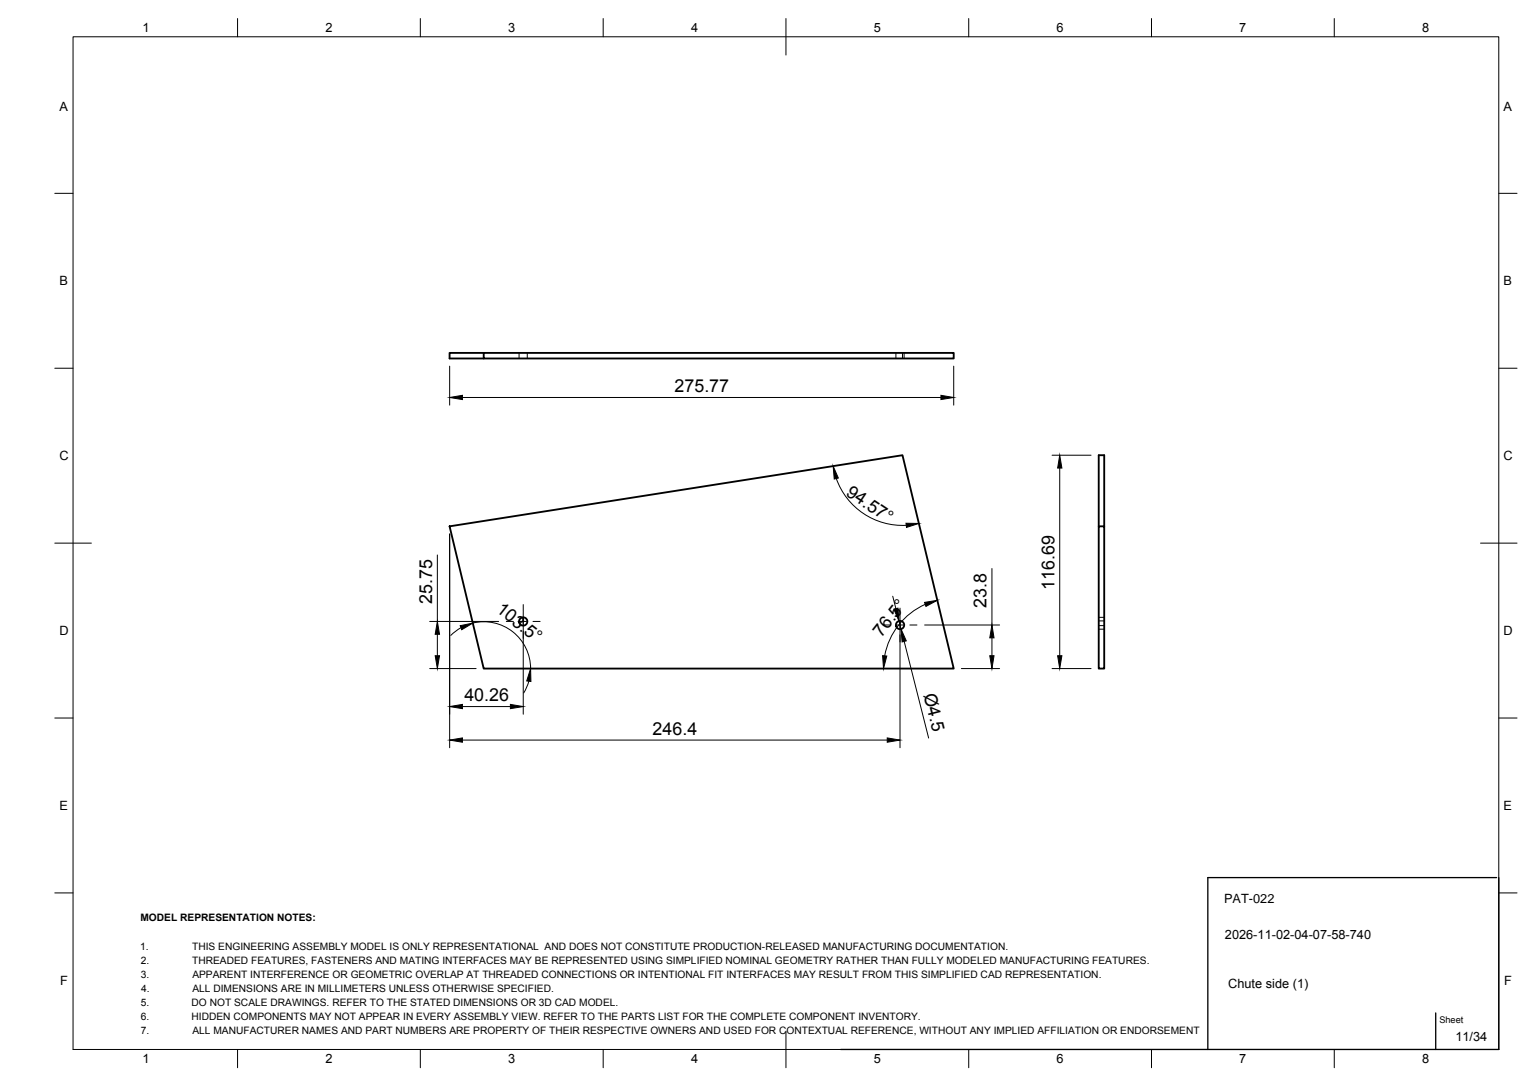
ISO-10303-21;
HEADER;
/* Generated by software containing ST-Developer
 * from STEP Tools, Inc. (www.steptools.com) 
 */

FILE_DESCRIPTION(
/* description */ ('Chute with adjustable gate'),
/* implementation_level */ '2;1');

FILE_NAME(
/* name */ 'Chute side (1).step',
/* time_stamp */ '2026-10-27T10:52:28-07:00',
/* author */ (''),
/* organization */ (''),
/* preprocessor_version */ 'ST-DEVELOPER v20.2',
/* originating_system */ 'Autodesk Translation Framework v15.17.0.0',
/* authorisation */ '');

FILE_SCHEMA (('AUTOMOTIVE_DESIGN { 1 0 10303 214 3 1 1 }'));
ENDSEC;

DATA;
#10=MECHANICAL_DESIGN_GEOMETRIC_PRESENTATION_REPRESENTATION('',(#420),#13094);
#356=SHAPE_REPRESENTATION_RELATIONSHIP('SRR','None',#13257,#388);
#388=ADVANCED_BREP_SHAPE_REPRESENTATION('',(#452),#13066);
#420=STYLED_ITEM('',(#13509),#452);
#452=MANIFOLD_SOLID_BREP('Body1',#7603);
#496=FACE_BOUND('',#1408,.T.);
#497=FACE_BOUND('',#1409,.T.);
#498=FACE_BOUND('',#1411,.T.);
#499=FACE_BOUND('',#1412,.T.);
#630=PLANE('',#8071);
#631=PLANE('',#8072);
#632=PLANE('',#8073);
#633=PLANE('',#8074);
#634=PLANE('',#8075);
#635=PLANE('',#8076);
#964=FACE_OUTER_BOUND('',#1401,.T.);
#965=FACE_OUTER_BOUND('',#1402,.T.);
#966=FACE_OUTER_BOUND('',#1403,.T.);
#967=FACE_OUTER_BOUND('',#1404,.T.);
#968=FACE_OUTER_BOUND('',#1405,.T.);
#969=FACE_OUTER_BOUND('',#1406,.T.);
#970=FACE_OUTER_BOUND('',#1407,.T.);
#971=FACE_OUTER_BOUND('',#1410,.T.);
#1401=EDGE_LOOP('',(#5414,#5415,#5416,#5417));
#1402=EDGE_LOOP('',(#5418,#5419,#5420,#5421));
#1403=EDGE_LOOP('',(#5422,#5423,#5424,#5425));
#1404=EDGE_LOOP('',(#5426,#5427,#5428,#5429));
#1405=EDGE_LOOP('',(#5430,#5431,#5432,#5433));
#1406=EDGE_LOOP('',(#5434,#5435,#5436,#5437));
#1407=EDGE_LOOP('',(#5438,#5439,#5440,#5441));
#1408=EDGE_LOOP('',(#5442));
#1409=EDGE_LOOP('',(#5443));
#1410=EDGE_LOOP('',(#5444,#5445,#5446,#5447));
#1411=EDGE_LOOP('',(#5448));
#1412=EDGE_LOOP('',(#5449));
#1954=LINE('',#11152,#2731);
#1955=LINE('',#11158,#2732);
#1956=LINE('',#11163,#2733);
#1957=LINE('',#11165,#2734);
#1958=LINE('',#11167,#2735);
#1959=LINE('',#11168,#2736);
#1960=LINE('',#11171,#2737);
#1961=LINE('',#11173,#2738);
#1962=LINE('',#11174,#2739);
#1963=LINE('',#11177,#2740);
#1964=LINE('',#11179,#2741);
#1965=LINE('',#11180,#2742);
#1966=LINE('',#11182,#2743);
#1967=LINE('',#11183,#2744);
#2731=VECTOR('',#8954,0.225);
#2732=VECTOR('',#8961,0.225000000000001);
#2733=VECTOR('',#8966,1.);
#2734=VECTOR('',#8967,1.);
#2735=VECTOR('',#8968,1.);
#2736=VECTOR('',#8969,1.);
#2737=VECTOR('',#8972,1.);
#2738=VECTOR('',#8973,1.);
#2739=VECTOR('',#8974,1.);
#2740=VECTOR('',#8977,1.);
#2741=VECTOR('',#8978,1.);
#2742=VECTOR('',#8979,1.);
#2743=VECTOR('',#8982,1.);
#2744=VECTOR('',#8983,1.);
#3434=CIRCLE('',#8066,0.225);
#3435=CIRCLE('',#8067,0.225);
#3436=CIRCLE('',#8069,0.225000000000001);
#3437=CIRCLE('',#8070,0.225000000000001);
#3669=VERTEX_POINT('',#11149);
#3670=VERTEX_POINT('',#11151);
#3671=VERTEX_POINT('',#11155);
#3672=VERTEX_POINT('',#11157);
#3673=VERTEX_POINT('',#11161);
#3674=VERTEX_POINT('',#11162);
#3675=VERTEX_POINT('',#11164);
#3676=VERTEX_POINT('',#11166);
#3677=VERTEX_POINT('',#11170);
#3678=VERTEX_POINT('',#11172);
#3679=VERTEX_POINT('',#11176);
#3680=VERTEX_POINT('',#11178);
#4340=EDGE_CURVE('',#3669,#3669,#3434,.T.);
#4341=EDGE_CURVE('',#3669,#3670,#1954,.T.);
#4342=EDGE_CURVE('',#3670,#3670,#3435,.T.);
#4343=EDGE_CURVE('',#3671,#3671,#3436,.T.);
#4344=EDGE_CURVE('',#3671,#3672,#1955,.T.);
#4345=EDGE_CURVE('',#3672,#3672,#3437,.T.);
#4346=EDGE_CURVE('',#3673,#3674,#1956,.T.);
#4347=EDGE_CURVE('',#3673,#3675,#1957,.T.);
#4348=EDGE_CURVE('',#3676,#3675,#1958,.T.);
#4349=EDGE_CURVE('',#3674,#3676,#1959,.T.);
#4350=EDGE_CURVE('',#3674,#3677,#1960,.T.);
#4351=EDGE_CURVE('',#3678,#3676,#1961,.T.);
#4352=EDGE_CURVE('',#3677,#3678,#1962,.T.);
#4353=EDGE_CURVE('',#3677,#3679,#1963,.T.);
#4354=EDGE_CURVE('',#3680,#3678,#1964,.T.);
#4355=EDGE_CURVE('',#3679,#3680,#1965,.T.);
#4356=EDGE_CURVE('',#3679,#3673,#1966,.T.);
#4357=EDGE_CURVE('',#3675,#3680,#1967,.T.);
#5414=ORIENTED_EDGE('',*,*,#4340,.F.);
#5415=ORIENTED_EDGE('',*,*,#4341,.T.);
#5416=ORIENTED_EDGE('',*,*,#4342,.F.);
#5417=ORIENTED_EDGE('',*,*,#4341,.F.);
#5418=ORIENTED_EDGE('',*,*,#4343,.F.);
#5419=ORIENTED_EDGE('',*,*,#4344,.T.);
#5420=ORIENTED_EDGE('',*,*,#4345,.F.);
#5421=ORIENTED_EDGE('',*,*,#4344,.F.);
#5422=ORIENTED_EDGE('',*,*,#4346,.F.);
#5423=ORIENTED_EDGE('',*,*,#4347,.T.);
#5424=ORIENTED_EDGE('',*,*,#4348,.F.);
#5425=ORIENTED_EDGE('',*,*,#4349,.F.);
#5426=ORIENTED_EDGE('',*,*,#4350,.F.);
#5427=ORIENTED_EDGE('',*,*,#4349,.T.);
#5428=ORIENTED_EDGE('',*,*,#4351,.F.);
#5429=ORIENTED_EDGE('',*,*,#4352,.F.);
#5430=ORIENTED_EDGE('',*,*,#4353,.F.);
#5431=ORIENTED_EDGE('',*,*,#4352,.T.);
#5432=ORIENTED_EDGE('',*,*,#4354,.F.);
#5433=ORIENTED_EDGE('',*,*,#4355,.F.);
#5434=ORIENTED_EDGE('',*,*,#4356,.F.);
#5435=ORIENTED_EDGE('',*,*,#4355,.T.);
#5436=ORIENTED_EDGE('',*,*,#4357,.F.);
#5437=ORIENTED_EDGE('',*,*,#4347,.F.);
#5438=ORIENTED_EDGE('',*,*,#4357,.T.);
#5439=ORIENTED_EDGE('',*,*,#4354,.T.);
#5440=ORIENTED_EDGE('',*,*,#4351,.T.);
#5441=ORIENTED_EDGE('',*,*,#4348,.T.);
#5442=ORIENTED_EDGE('',*,*,#4342,.T.);
#5443=ORIENTED_EDGE('',*,*,#4345,.T.);
#5444=ORIENTED_EDGE('',*,*,#4356,.T.);
#5445=ORIENTED_EDGE('',*,*,#4346,.T.);
#5446=ORIENTED_EDGE('',*,*,#4350,.T.);
#5447=ORIENTED_EDGE('',*,*,#4353,.T.);
#5448=ORIENTED_EDGE('',*,*,#4340,.T.);
#5449=ORIENTED_EDGE('',*,*,#4343,.T.);
#7116=CYLINDRICAL_SURFACE('',#8065,0.225);
#7117=CYLINDRICAL_SURFACE('',#8068,0.225000000000001);
#7232=ADVANCED_FACE('',(#964),#7116,.F.);
#7233=ADVANCED_FACE('',(#965),#7117,.F.);
#7234=ADVANCED_FACE('',(#966),#630,.T.);
#7235=ADVANCED_FACE('',(#967),#631,.T.);
#7236=ADVANCED_FACE('',(#968),#632,.T.);
#7237=ADVANCED_FACE('',(#969),#633,.T.);
#7238=ADVANCED_FACE('',(#970,#496,#497),#634,.T.);
#7239=ADVANCED_FACE('',(#971,#498,#499),#635,.F.);
#7603=CLOSED_SHELL('',(#7232,#7233,#7234,#7235,#7236,#7237,#7238,#7239));
#8064=AXIS2_PLACEMENT_3D('',#11147,#8948,#8949);
#8065=AXIS2_PLACEMENT_3D('',#11148,#8950,#8951);
#8066=AXIS2_PLACEMENT_3D('',#11150,#8952,#8953);
#8067=AXIS2_PLACEMENT_3D('',#11153,#8955,#8956);
#8068=AXIS2_PLACEMENT_3D('',#11154,#8957,#8958);
#8069=AXIS2_PLACEMENT_3D('',#11156,#8959,#8960);
#8070=AXIS2_PLACEMENT_3D('',#11159,#8962,#8963);
#8071=AXIS2_PLACEMENT_3D('',#11160,#8964,#8965);
#8072=AXIS2_PLACEMENT_3D('',#11169,#8970,#8971);
#8073=AXIS2_PLACEMENT_3D('',#11175,#8975,#8976);
#8074=AXIS2_PLACEMENT_3D('',#11181,#8980,#8981);
#8075=AXIS2_PLACEMENT_3D('',#11184,#8984,#8985);
#8076=AXIS2_PLACEMENT_3D('',#11185,#8986,#8987);
#8948=DIRECTION('axis',(0.,0.,1.));
#8949=DIRECTION('refdir',(1.,0.,0.));
#8950=DIRECTION('center_axis',(0.,1.,0.));
#8951=DIRECTION('ref_axis',(1.,0.,0.));
#8952=DIRECTION('center_axis',(0.,1.,0.));
#8953=DIRECTION('ref_axis',(1.,0.,0.));
#8954=DIRECTION('',(0.,1.,0.));
#8955=DIRECTION('center_axis',(0.,-1.,0.));
#8956=DIRECTION('ref_axis',(1.,0.,0.));
#8957=DIRECTION('center_axis',(0.,1.,0.));
#8958=DIRECTION('ref_axis',(1.,0.,0.));
#8959=DIRECTION('center_axis',(0.,1.,0.));
#8960=DIRECTION('ref_axis',(1.,0.,0.));
#8961=DIRECTION('',(0.,1.,0.));
#8962=DIRECTION('center_axis',(0.,-1.,0.));
#8963=DIRECTION('ref_axis',(1.,0.,0.));
#8964=DIRECTION('center_axis',(-1.,0.,0.));
#8965=DIRECTION('ref_axis',(0.,0.,1.));
#8966=DIRECTION('',(0.,0.,-1.));
#8967=DIRECTION('',(0.,1.,0.));
#8968=DIRECTION('',(0.,0.,1.));
#8969=DIRECTION('',(0.,1.,0.));
#8970=DIRECTION('center_axis',(0.233372952475324,0.,-0.972387301980517));
#8971=DIRECTION('ref_axis',(-0.972387301980517,0.,-0.233372952475324));
#8972=DIRECTION('',(0.972387301980517,0.,0.233372952475324));
#8973=DIRECTION('',(-0.972387301980517,0.,-0.233372952475324));
#8974=DIRECTION('',(0.,1.,0.));
#8975=DIRECTION('center_axis',(1.,0.,0.));
#8976=DIRECTION('ref_axis',(0.,0.,-1.));
#8977=DIRECTION('',(0.,0.,1.));
#8978=DIRECTION('',(0.,0.,-1.));
#8979=DIRECTION('',(0.,1.,0.));
#8980=DIRECTION('center_axis',(-0.07974522228289,0.,0.996815278536125));
#8981=DIRECTION('ref_axis',(0.996815278536125,0.,0.07974522228289));
#8982=DIRECTION('',(-0.996815278536125,0.,-0.07974522228289));
#8983=DIRECTION('',(0.996815278536125,0.,0.07974522228289));
#8984=DIRECTION('center_axis',(0.,1.,0.));
#8985=DIRECTION('ref_axis',(0.,0.,1.));
#8986=DIRECTION('center_axis',(0.,1.,0.));
#8987=DIRECTION('ref_axis',(1.,0.,0.));
#11147=CARTESIAN_POINT('',(0.,0.,0.));
#11148=CARTESIAN_POINT('Origin',(2.3,7.4,7.));
#11149=CARTESIAN_POINT('',(2.075,7.5,7.));
#11150=CARTESIAN_POINT('Origin',(2.3,7.5,7.));
#11151=CARTESIAN_POINT('',(2.075,7.8,7.));
#11152=CARTESIAN_POINT('',(2.075,7.4,7.));
#11153=CARTESIAN_POINT('Origin',(2.3,7.8,7.));
#11154=CARTESIAN_POINT('Origin',(22.3,7.4,12.));
#11155=CARTESIAN_POINT('',(22.075,7.5,12.));
#11156=CARTESIAN_POINT('Origin',(22.3,7.5,12.));
#11157=CARTESIAN_POINT('',(22.075,7.8,12.));
#11158=CARTESIAN_POINT('',(22.075,7.4,12.));
#11159=CARTESIAN_POINT('Origin',(22.3,7.8,12.));
#11160=CARTESIAN_POINT('Origin',(0.,7.5,4.));
#11161=CARTESIAN_POINT('',(0.,7.5,16.));
#11162=CARTESIAN_POINT('',(0.,7.5,4.));
#11163=CARTESIAN_POINT('',(0.,7.5,16.));
#11164=CARTESIAN_POINT('',(0.,7.8,16.));
#11165=CARTESIAN_POINT('',(0.,7.5,16.));
#11166=CARTESIAN_POINT('',(0.,7.8,4.));
#11167=CARTESIAN_POINT('',(0.,7.8,16.));
#11168=CARTESIAN_POINT('',(0.,7.5,4.));
#11169=CARTESIAN_POINT('Origin',(25.,7.5,10.));
#11170=CARTESIAN_POINT('',(25.,7.5,10.));
#11171=CARTESIAN_POINT('',(0.,7.5,4.));
#11172=CARTESIAN_POINT('',(25.,7.8,10.));
#11173=CARTESIAN_POINT('',(0.,7.8,4.));
#11174=CARTESIAN_POINT('',(25.,7.5,10.));
#11175=CARTESIAN_POINT('Origin',(25.,7.5,18.));
#11176=CARTESIAN_POINT('',(25.,7.5,18.));
#11177=CARTESIAN_POINT('',(25.,7.5,10.));
#11178=CARTESIAN_POINT('',(25.,7.8,18.));
#11179=CARTESIAN_POINT('',(25.,7.8,10.));
#11180=CARTESIAN_POINT('',(25.,7.5,18.));
#11181=CARTESIAN_POINT('Origin',(0.,7.5,16.));
#11182=CARTESIAN_POINT('',(25.,7.5,18.));
#11183=CARTESIAN_POINT('',(25.,7.8,18.));
#11184=CARTESIAN_POINT('Origin',(12.5,7.8,11.));
#11185=CARTESIAN_POINT('Origin',(12.5,7.5,11.));
#13029=UNCERTAINTY_MEASURE_WITH_UNIT(LENGTH_MEASURE(0.001),#13095,
'DISTANCE_ACCURACY_VALUE',
'Maximum model space distance between geometric entities at asserted c
onnectivities');
#13057=UNCERTAINTY_MEASURE_WITH_UNIT(LENGTH_MEASURE(0.001),#13095,
'DISTANCE_ACCURACY_VALUE',
'Maximum model space distance between geometric entities at asserted c
onnectivities');
#13066=(
GEOMETRIC_REPRESENTATION_CONTEXT(3)
GLOBAL_UNCERTAINTY_ASSIGNED_CONTEXT((#13029))
GLOBAL_UNIT_ASSIGNED_CONTEXT((#13095,#13097,#13098))
REPRESENTATION_CONTEXT('','3D')
);
#13094=(
GEOMETRIC_REPRESENTATION_CONTEXT(3)
GLOBAL_UNCERTAINTY_ASSIGNED_CONTEXT((#13057))
GLOBAL_UNIT_ASSIGNED_CONTEXT((#13095,#13097,#13098))
REPRESENTATION_CONTEXT('','3D')
);
#13095=(
LENGTH_UNIT()
NAMED_UNIT(*)
SI_UNIT(.CENTI.,.METRE.)
);
#13097=(
NAMED_UNIT(*)
PLANE_ANGLE_UNIT()
SI_UNIT($,.RADIAN.)
);
#13098=(
NAMED_UNIT(*)
SI_UNIT($,.STERADIAN.)
SOLID_ANGLE_UNIT()
);
#13107=SHAPE_DEFINITION_REPRESENTATION(#13143,#13257);
#13143=PRODUCT_DEFINITION_SHAPE('',$,#13294);
#13257=SHAPE_REPRESENTATION('',(#8064),#13066);
#13285=PRODUCT_DEFINITION_CONTEXT('part definition',#13395,'design');
#13294=PRODUCT_DEFINITION('Chute side (1)','Chute side (1)',#13330,#13285);
#13330=PRODUCT_DEFINITION_FORMATION('',$,#13405);
#13395=APPLICATION_CONTEXT(
'Core Data for Automotive Mechanical Design Process');
#13396=PRODUCT_CONTEXT('part definition',#13395,'mechanical');
#13405=PRODUCT('Chute side (1)','Chute side (1)','Chute side (1)',(#13396));
#13503=COLOUR_RGB('Off White',0.89,0.88,0.83);
#13504=FILL_AREA_STYLE_COLOUR('',#13503);
#13505=FILL_AREA_STYLE('',(#13504));
#13506=SURFACE_STYLE_FILL_AREA(#13505);
#13507=SURFACE_SIDE_STYLE('',(#13506));
#13508=SURFACE_STYLE_USAGE(.BOTH.,#13507);
#13509=PRESENTATION_STYLE_ASSIGNMENT((#13508));
ENDSEC;
END-ISO-10303-21;
